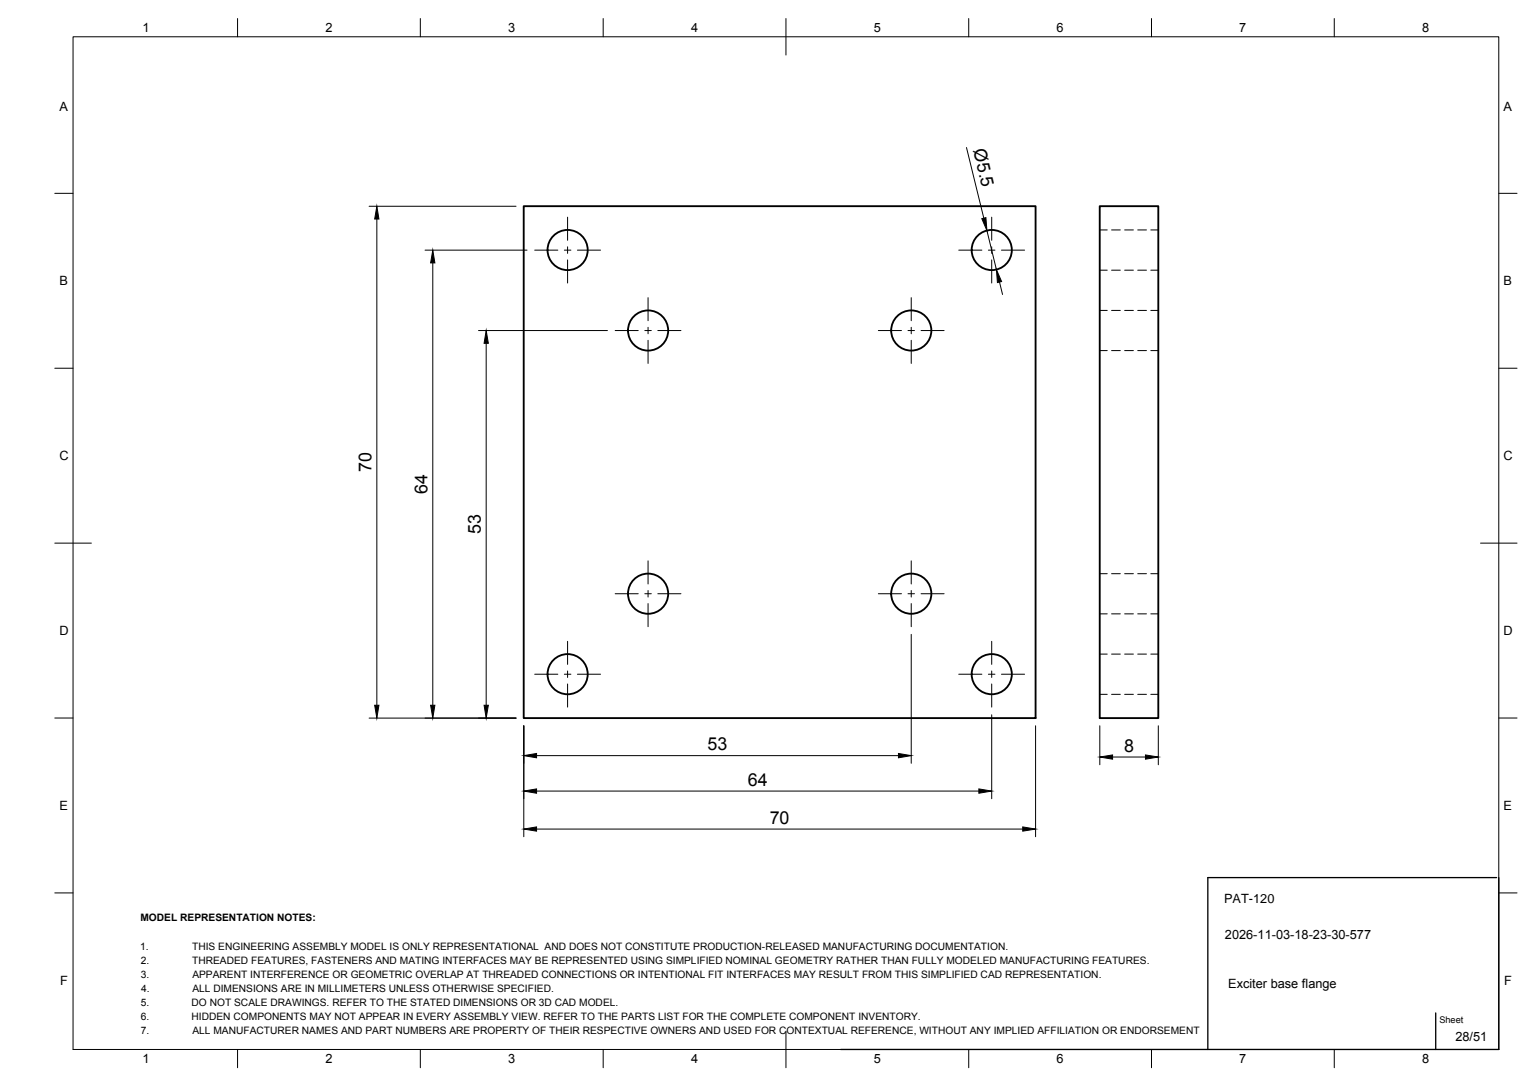
ISO-10303-21;
HEADER;
/* Generated by software containing ST-Developer
 * from STEP Tools, Inc. (www.steptools.com) 
 */

FILE_DESCRIPTION(
/* description */ ('Vibration shaker table dummy'),
/* implementation_level */ '2;1');

FILE_NAME(
/* name */ 'Exciter base flange.step',
/* time_stamp */ '2026-10-27T10:55:14-07:00',
/* author */ (''),
/* organization */ (''),
/* preprocessor_version */ 'ST-DEVELOPER v20.2',
/* originating_system */ 'Autodesk Translation Framework v15.17.0.0',
/* authorisation */ '');

FILE_SCHEMA (('AUTOMOTIVE_DESIGN { 1 0 10303 214 3 1 1 }'));
ENDSEC;

DATA;
#10=MECHANICAL_DESIGN_GEOMETRIC_PRESENTATION_REPRESENTATION('',(#709),#22394);
#617=SHAPE_REPRESENTATION_RELATIONSHIP('SRR','None',#22663,#663);
#663=ADVANCED_BREP_SHAPE_REPRESENTATION('',(#755),#22369);
#709=STYLED_ITEM('',(#22940),#755);
#755=MANIFOLD_SOLID_BREP('Body1',#9227);
#925=FACE_BOUND('',#2244,.T.);
#926=FACE_BOUND('',#2245,.T.);
#927=FACE_BOUND('',#2246,.T.);
#928=FACE_BOUND('',#2247,.T.);
#929=FACE_BOUND('',#2248,.T.);
#930=FACE_BOUND('',#2249,.T.);
#931=FACE_BOUND('',#2250,.T.);
#932=FACE_BOUND('',#2251,.T.);
#933=FACE_BOUND('',#2253,.T.);
#934=FACE_BOUND('',#2254,.T.);
#935=FACE_BOUND('',#2255,.T.);
#936=FACE_BOUND('',#2256,.T.);
#937=FACE_BOUND('',#2257,.T.);
#938=FACE_BOUND('',#2258,.T.);
#939=FACE_BOUND('',#2259,.T.);
#940=FACE_BOUND('',#2260,.T.);
#1204=PLANE('',#10260);
#1205=PLANE('',#10261);
#1206=PLANE('',#10262);
#1207=PLANE('',#10263);
#1208=PLANE('',#10264);
#1209=PLANE('',#10265);
#1583=FACE_OUTER_BOUND('',#2231,.T.);
#1584=FACE_OUTER_BOUND('',#2232,.T.);
#1585=FACE_OUTER_BOUND('',#2233,.T.);
#1586=FACE_OUTER_BOUND('',#2234,.T.);
#1587=FACE_OUTER_BOUND('',#2235,.T.);
#1588=FACE_OUTER_BOUND('',#2236,.T.);
#1589=FACE_OUTER_BOUND('',#2237,.T.);
#1590=FACE_OUTER_BOUND('',#2238,.T.);
#1591=FACE_OUTER_BOUND('',#2239,.T.);
#1592=FACE_OUTER_BOUND('',#2240,.T.);
#1593=FACE_OUTER_BOUND('',#2241,.T.);
#1594=FACE_OUTER_BOUND('',#2242,.T.);
#1595=FACE_OUTER_BOUND('',#2243,.T.);
#1596=FACE_OUTER_BOUND('',#2252,.T.);
#2231=EDGE_LOOP('',(#7338,#7339,#7340,#7341));
#2232=EDGE_LOOP('',(#7342,#7343,#7344,#7345));
#2233=EDGE_LOOP('',(#7346,#7347,#7348,#7349));
#2234=EDGE_LOOP('',(#7350,#7351,#7352,#7353));
#2235=EDGE_LOOP('',(#7354,#7355,#7356,#7357));
#2236=EDGE_LOOP('',(#7358,#7359,#7360,#7361));
#2237=EDGE_LOOP('',(#7362,#7363,#7364,#7365));
#2238=EDGE_LOOP('',(#7366,#7367,#7368,#7369));
#2239=EDGE_LOOP('',(#7370,#7371,#7372,#7373));
#2240=EDGE_LOOP('',(#7374,#7375,#7376,#7377));
#2241=EDGE_LOOP('',(#7378,#7379,#7380,#7381));
#2242=EDGE_LOOP('',(#7382,#7383,#7384,#7385));
#2243=EDGE_LOOP('',(#7386,#7387,#7388,#7389));
#2244=EDGE_LOOP('',(#7390));
#2245=EDGE_LOOP('',(#7391));
#2246=EDGE_LOOP('',(#7392));
#2247=EDGE_LOOP('',(#7393));
#2248=EDGE_LOOP('',(#7394));
#2249=EDGE_LOOP('',(#7395));
#2250=EDGE_LOOP('',(#7396));
#2251=EDGE_LOOP('',(#7397));
#2252=EDGE_LOOP('',(#7398,#7399,#7400,#7401));
#2253=EDGE_LOOP('',(#7402));
#2254=EDGE_LOOP('',(#7403));
#2255=EDGE_LOOP('',(#7404));
#2256=EDGE_LOOP('',(#7405));
#2257=EDGE_LOOP('',(#7406));
#2258=EDGE_LOOP('',(#7407));
#2259=EDGE_LOOP('',(#7408));
#2260=EDGE_LOOP('',(#7409));
#2952=LINE('',#20909,#3571);
#2953=LINE('',#20915,#3572);
#2954=LINE('',#20921,#3573);
#2955=LINE('',#20927,#3574);
#2956=LINE('',#20933,#3575);
#2957=LINE('',#20939,#3576);
#2958=LINE('',#20945,#3577);
#2959=LINE('',#20951,#3578);
#2960=LINE('',#20956,#3579);
#2961=LINE('',#20958,#3580);
#2962=LINE('',#20960,#3581);
#2963=LINE('',#20961,#3582);
#2964=LINE('',#20964,#3583);
#2965=LINE('',#20966,#3584);
#2966=LINE('',#20967,#3585);
#2967=LINE('',#20970,#3586);
#2968=LINE('',#20972,#3587);
#2969=LINE('',#20973,#3588);
#2970=LINE('',#20975,#3589);
#2971=LINE('',#20976,#3590);
#3571=VECTOR('',#12236,0.275);
#3572=VECTOR('',#12243,0.275);
#3573=VECTOR('',#12250,0.275);
#3574=VECTOR('',#12257,0.275);
#3575=VECTOR('',#12264,0.275);
#3576=VECTOR('',#12271,0.275);
#3577=VECTOR('',#12278,0.275);
#3578=VECTOR('',#12285,0.275);
#3579=VECTOR('',#12290,1.);
#3580=VECTOR('',#12291,1.);
#3581=VECTOR('',#12292,1.);
#3582=VECTOR('',#12293,1.);
#3583=VECTOR('',#12296,1.);
#3584=VECTOR('',#12297,1.);
#3585=VECTOR('',#12298,1.);
#3586=VECTOR('',#12301,1.);
#3587=VECTOR('',#12302,1.);
#3588=VECTOR('',#12303,1.);
#3589=VECTOR('',#12306,1.);
#3590=VECTOR('',#12307,1.);
#4072=CIRCLE('',#10237,0.275);
#4073=CIRCLE('',#10238,0.275);
#4074=CIRCLE('',#10240,0.275);
#4075=CIRCLE('',#10241,0.275);
#4076=CIRCLE('',#10243,0.275);
#4077=CIRCLE('',#10244,0.275);
#4078=CIRCLE('',#10246,0.275);
#4079=CIRCLE('',#10247,0.275);
#4080=CIRCLE('',#10249,0.275);
#4081=CIRCLE('',#10250,0.275);
#4082=CIRCLE('',#10252,0.275);
#4083=CIRCLE('',#10253,0.275);
#4084=CIRCLE('',#10255,0.275);
#4085=CIRCLE('',#10256,0.275);
#4086=CIRCLE('',#10258,0.275);
#4087=CIRCLE('',#10259,0.275);
#4731=VERTEX_POINT('',#20906);
#4732=VERTEX_POINT('',#20908);
#4733=VERTEX_POINT('',#20912);
#4734=VERTEX_POINT('',#20914);
#4735=VERTEX_POINT('',#20918);
#4736=VERTEX_POINT('',#20920);
#4737=VERTEX_POINT('',#20924);
#4738=VERTEX_POINT('',#20926);
#4739=VERTEX_POINT('',#20930);
#4740=VERTEX_POINT('',#20932);
#4741=VERTEX_POINT('',#20936);
#4742=VERTEX_POINT('',#20938);
#4743=VERTEX_POINT('',#20942);
#4744=VERTEX_POINT('',#20944);
#4745=VERTEX_POINT('',#20948);
#4746=VERTEX_POINT('',#20950);
#4747=VERTEX_POINT('',#20954);
#4748=VERTEX_POINT('',#20955);
#4749=VERTEX_POINT('',#20957);
#4750=VERTEX_POINT('',#20959);
#4751=VERTEX_POINT('',#20963);
#4752=VERTEX_POINT('',#20965);
#4753=VERTEX_POINT('',#20969);
#4754=VERTEX_POINT('',#20971);
#5662=EDGE_CURVE('',#4731,#4731,#4072,.T.);
#5663=EDGE_CURVE('',#4731,#4732,#2952,.T.);
#5664=EDGE_CURVE('',#4732,#4732,#4073,.T.);
#5665=EDGE_CURVE('',#4733,#4733,#4074,.T.);
#5666=EDGE_CURVE('',#4733,#4734,#2953,.T.);
#5667=EDGE_CURVE('',#4734,#4734,#4075,.T.);
#5668=EDGE_CURVE('',#4735,#4735,#4076,.T.);
#5669=EDGE_CURVE('',#4735,#4736,#2954,.T.);
#5670=EDGE_CURVE('',#4736,#4736,#4077,.T.);
#5671=EDGE_CURVE('',#4737,#4737,#4078,.T.);
#5672=EDGE_CURVE('',#4737,#4738,#2955,.T.);
#5673=EDGE_CURVE('',#4738,#4738,#4079,.T.);
#5674=EDGE_CURVE('',#4739,#4739,#4080,.T.);
#5675=EDGE_CURVE('',#4739,#4740,#2956,.T.);
#5676=EDGE_CURVE('',#4740,#4740,#4081,.T.);
#5677=EDGE_CURVE('',#4741,#4741,#4082,.T.);
#5678=EDGE_CURVE('',#4741,#4742,#2957,.T.);
#5679=EDGE_CURVE('',#4742,#4742,#4083,.T.);
#5680=EDGE_CURVE('',#4743,#4743,#4084,.T.);
#5681=EDGE_CURVE('',#4743,#4744,#2958,.T.);
#5682=EDGE_CURVE('',#4744,#4744,#4085,.T.);
#5683=EDGE_CURVE('',#4745,#4745,#4086,.T.);
#5684=EDGE_CURVE('',#4745,#4746,#2959,.T.);
#5685=EDGE_CURVE('',#4746,#4746,#4087,.T.);
#5686=EDGE_CURVE('',#4747,#4748,#2960,.T.);
#5687=EDGE_CURVE('',#4748,#4749,#2961,.T.);
#5688=EDGE_CURVE('',#4750,#4749,#2962,.T.);
#5689=EDGE_CURVE('',#4747,#4750,#2963,.T.);
#5690=EDGE_CURVE('',#4751,#4747,#2964,.T.);
#5691=EDGE_CURVE('',#4752,#4750,#2965,.T.);
#5692=EDGE_CURVE('',#4751,#4752,#2966,.T.);
#5693=EDGE_CURVE('',#4753,#4751,#2967,.T.);
#5694=EDGE_CURVE('',#4754,#4752,#2968,.T.);
#5695=EDGE_CURVE('',#4753,#4754,#2969,.T.);
#5696=EDGE_CURVE('',#4748,#4753,#2970,.T.);
#5697=EDGE_CURVE('',#4749,#4754,#2971,.T.);
#7338=ORIENTED_EDGE('',*,*,#5662,.F.);
#7339=ORIENTED_EDGE('',*,*,#5663,.T.);
#7340=ORIENTED_EDGE('',*,*,#5664,.F.);
#7341=ORIENTED_EDGE('',*,*,#5663,.F.);
#7342=ORIENTED_EDGE('',*,*,#5665,.F.);
#7343=ORIENTED_EDGE('',*,*,#5666,.T.);
#7344=ORIENTED_EDGE('',*,*,#5667,.F.);
#7345=ORIENTED_EDGE('',*,*,#5666,.F.);
#7346=ORIENTED_EDGE('',*,*,#5668,.F.);
#7347=ORIENTED_EDGE('',*,*,#5669,.T.);
#7348=ORIENTED_EDGE('',*,*,#5670,.F.);
#7349=ORIENTED_EDGE('',*,*,#5669,.F.);
#7350=ORIENTED_EDGE('',*,*,#5671,.F.);
#7351=ORIENTED_EDGE('',*,*,#5672,.T.);
#7352=ORIENTED_EDGE('',*,*,#5673,.F.);
#7353=ORIENTED_EDGE('',*,*,#5672,.F.);
#7354=ORIENTED_EDGE('',*,*,#5674,.F.);
#7355=ORIENTED_EDGE('',*,*,#5675,.T.);
#7356=ORIENTED_EDGE('',*,*,#5676,.F.);
#7357=ORIENTED_EDGE('',*,*,#5675,.F.);
#7358=ORIENTED_EDGE('',*,*,#5677,.F.);
#7359=ORIENTED_EDGE('',*,*,#5678,.T.);
#7360=ORIENTED_EDGE('',*,*,#5679,.F.);
#7361=ORIENTED_EDGE('',*,*,#5678,.F.);
#7362=ORIENTED_EDGE('',*,*,#5680,.F.);
#7363=ORIENTED_EDGE('',*,*,#5681,.T.);
#7364=ORIENTED_EDGE('',*,*,#5682,.F.);
#7365=ORIENTED_EDGE('',*,*,#5681,.F.);
#7366=ORIENTED_EDGE('',*,*,#5683,.F.);
#7367=ORIENTED_EDGE('',*,*,#5684,.T.);
#7368=ORIENTED_EDGE('',*,*,#5685,.F.);
#7369=ORIENTED_EDGE('',*,*,#5684,.F.);
#7370=ORIENTED_EDGE('',*,*,#5686,.T.);
#7371=ORIENTED_EDGE('',*,*,#5687,.T.);
#7372=ORIENTED_EDGE('',*,*,#5688,.F.);
#7373=ORIENTED_EDGE('',*,*,#5689,.F.);
#7374=ORIENTED_EDGE('',*,*,#5690,.T.);
#7375=ORIENTED_EDGE('',*,*,#5689,.T.);
#7376=ORIENTED_EDGE('',*,*,#5691,.F.);
#7377=ORIENTED_EDGE('',*,*,#5692,.F.);
#7378=ORIENTED_EDGE('',*,*,#5693,.T.);
#7379=ORIENTED_EDGE('',*,*,#5692,.T.);
#7380=ORIENTED_EDGE('',*,*,#5694,.F.);
#7381=ORIENTED_EDGE('',*,*,#5695,.F.);
#7382=ORIENTED_EDGE('',*,*,#5696,.T.);
#7383=ORIENTED_EDGE('',*,*,#5695,.T.);
#7384=ORIENTED_EDGE('',*,*,#5697,.F.);
#7385=ORIENTED_EDGE('',*,*,#5687,.F.);
#7386=ORIENTED_EDGE('',*,*,#5697,.T.);
#7387=ORIENTED_EDGE('',*,*,#5694,.T.);
#7388=ORIENTED_EDGE('',*,*,#5691,.T.);
#7389=ORIENTED_EDGE('',*,*,#5688,.T.);
#7390=ORIENTED_EDGE('',*,*,#5685,.T.);
#7391=ORIENTED_EDGE('',*,*,#5682,.T.);
#7392=ORIENTED_EDGE('',*,*,#5679,.T.);
#7393=ORIENTED_EDGE('',*,*,#5676,.T.);
#7394=ORIENTED_EDGE('',*,*,#5673,.T.);
#7395=ORIENTED_EDGE('',*,*,#5670,.T.);
#7396=ORIENTED_EDGE('',*,*,#5667,.T.);
#7397=ORIENTED_EDGE('',*,*,#5664,.T.);
#7398=ORIENTED_EDGE('',*,*,#5696,.F.);
#7399=ORIENTED_EDGE('',*,*,#5686,.F.);
#7400=ORIENTED_EDGE('',*,*,#5690,.F.);
#7401=ORIENTED_EDGE('',*,*,#5693,.F.);
#7402=ORIENTED_EDGE('',*,*,#5683,.T.);
#7403=ORIENTED_EDGE('',*,*,#5680,.T.);
#7404=ORIENTED_EDGE('',*,*,#5677,.T.);
#7405=ORIENTED_EDGE('',*,*,#5674,.T.);
#7406=ORIENTED_EDGE('',*,*,#5671,.T.);
#7407=ORIENTED_EDGE('',*,*,#5668,.T.);
#7408=ORIENTED_EDGE('',*,*,#5665,.T.);
#7409=ORIENTED_EDGE('',*,*,#5662,.T.);
#8600=CYLINDRICAL_SURFACE('',#10236,0.275);
#8601=CYLINDRICAL_SURFACE('',#10239,0.275);
#8602=CYLINDRICAL_SURFACE('',#10242,0.275);
#8603=CYLINDRICAL_SURFACE('',#10245,0.275);
#8604=CYLINDRICAL_SURFACE('',#10248,0.275);
#8605=CYLINDRICAL_SURFACE('',#10251,0.275);
#8606=CYLINDRICAL_SURFACE('',#10254,0.275);
#8607=CYLINDRICAL_SURFACE('',#10257,0.275);
#8948=ADVANCED_FACE('',(#1583),#8600,.F.);
#8949=ADVANCED_FACE('',(#1584),#8601,.F.);
#8950=ADVANCED_FACE('',(#1585),#8602,.F.);
#8951=ADVANCED_FACE('',(#1586),#8603,.F.);
#8952=ADVANCED_FACE('',(#1587),#8604,.F.);
#8953=ADVANCED_FACE('',(#1588),#8605,.F.);
#8954=ADVANCED_FACE('',(#1589),#8606,.F.);
#8955=ADVANCED_FACE('',(#1590),#8607,.F.);
#8956=ADVANCED_FACE('',(#1591),#1204,.T.);
#8957=ADVANCED_FACE('',(#1592),#1205,.T.);
#8958=ADVANCED_FACE('',(#1593),#1206,.T.);
#8959=ADVANCED_FACE('',(#1594),#1207,.T.);
#8960=ADVANCED_FACE('',(#1595,#925,#926,#927,#928,#929,#930,#931,#932),
#1208,.T.);
#8961=ADVANCED_FACE('',(#1596,#933,#934,#935,#936,#937,#938,#939,#940),
#1209,.F.);
#9227=CLOSED_SHELL('',(#8948,#8949,#8950,#8951,#8952,#8953,#8954,#8955,
#8956,#8957,#8958,#8959,#8960,#8961));
#10235=AXIS2_PLACEMENT_3D('',#20904,#12230,#12231);
#10236=AXIS2_PLACEMENT_3D('',#20905,#12232,#12233);
#10237=AXIS2_PLACEMENT_3D('',#20907,#12234,#12235);
#10238=AXIS2_PLACEMENT_3D('',#20910,#12237,#12238);
#10239=AXIS2_PLACEMENT_3D('',#20911,#12239,#12240);
#10240=AXIS2_PLACEMENT_3D('',#20913,#12241,#12242);
#10241=AXIS2_PLACEMENT_3D('',#20916,#12244,#12245);
#10242=AXIS2_PLACEMENT_3D('',#20917,#12246,#12247);
#10243=AXIS2_PLACEMENT_3D('',#20919,#12248,#12249);
#10244=AXIS2_PLACEMENT_3D('',#20922,#12251,#12252);
#10245=AXIS2_PLACEMENT_3D('',#20923,#12253,#12254);
#10246=AXIS2_PLACEMENT_3D('',#20925,#12255,#12256);
#10247=AXIS2_PLACEMENT_3D('',#20928,#12258,#12259);
#10248=AXIS2_PLACEMENT_3D('',#20929,#12260,#12261);
#10249=AXIS2_PLACEMENT_3D('',#20931,#12262,#12263);
#10250=AXIS2_PLACEMENT_3D('',#20934,#12265,#12266);
#10251=AXIS2_PLACEMENT_3D('',#20935,#12267,#12268);
#10252=AXIS2_PLACEMENT_3D('',#20937,#12269,#12270);
#10253=AXIS2_PLACEMENT_3D('',#20940,#12272,#12273);
#10254=AXIS2_PLACEMENT_3D('',#20941,#12274,#12275);
#10255=AXIS2_PLACEMENT_3D('',#20943,#12276,#12277);
#10256=AXIS2_PLACEMENT_3D('',#20946,#12279,#12280);
#10257=AXIS2_PLACEMENT_3D('',#20947,#12281,#12282);
#10258=AXIS2_PLACEMENT_3D('',#20949,#12283,#12284);
#10259=AXIS2_PLACEMENT_3D('',#20952,#12286,#12287);
#10260=AXIS2_PLACEMENT_3D('',#20953,#12288,#12289);
#10261=AXIS2_PLACEMENT_3D('',#20962,#12294,#12295);
#10262=AXIS2_PLACEMENT_3D('',#20968,#12299,#12300);
#10263=AXIS2_PLACEMENT_3D('',#20974,#12304,#12305);
#10264=AXIS2_PLACEMENT_3D('',#20977,#12308,#12309);
#10265=AXIS2_PLACEMENT_3D('',#20978,#12310,#12311);
#12230=DIRECTION('axis',(0.,0.,1.));
#12231=DIRECTION('refdir',(1.,0.,0.));
#12232=DIRECTION('center_axis',(0.,0.,1.));
#12233=DIRECTION('ref_axis',(1.,0.,0.));
#12234=DIRECTION('center_axis',(0.,0.,1.));
#12235=DIRECTION('ref_axis',(1.,0.,0.));
#12236=DIRECTION('',(0.,0.,1.));
#12237=DIRECTION('center_axis',(0.,0.,-1.));
#12238=DIRECTION('ref_axis',(1.,0.,0.));
#12239=DIRECTION('center_axis',(0.,0.,1.));
#12240=DIRECTION('ref_axis',(1.,0.,0.));
#12241=DIRECTION('center_axis',(0.,0.,1.));
#12242=DIRECTION('ref_axis',(1.,0.,0.));
#12243=DIRECTION('',(0.,0.,1.));
#12244=DIRECTION('center_axis',(0.,0.,-1.));
#12245=DIRECTION('ref_axis',(1.,0.,0.));
#12246=DIRECTION('center_axis',(0.,0.,1.));
#12247=DIRECTION('ref_axis',(1.,0.,0.));
#12248=DIRECTION('center_axis',(0.,0.,1.));
#12249=DIRECTION('ref_axis',(1.,0.,0.));
#12250=DIRECTION('',(0.,0.,1.));
#12251=DIRECTION('center_axis',(0.,0.,-1.));
#12252=DIRECTION('ref_axis',(1.,0.,0.));
#12253=DIRECTION('center_axis',(0.,0.,1.));
#12254=DIRECTION('ref_axis',(1.,0.,0.));
#12255=DIRECTION('center_axis',(0.,0.,1.));
#12256=DIRECTION('ref_axis',(1.,0.,0.));
#12257=DIRECTION('',(0.,0.,1.));
#12258=DIRECTION('center_axis',(0.,0.,-1.));
#12259=DIRECTION('ref_axis',(1.,0.,0.));
#12260=DIRECTION('center_axis',(0.,0.,1.));
#12261=DIRECTION('ref_axis',(1.,0.,0.));
#12262=DIRECTION('center_axis',(0.,0.,1.));
#12263=DIRECTION('ref_axis',(1.,0.,0.));
#12264=DIRECTION('',(0.,0.,1.));
#12265=DIRECTION('center_axis',(0.,0.,-1.));
#12266=DIRECTION('ref_axis',(1.,0.,0.));
#12267=DIRECTION('center_axis',(0.,0.,1.));
#12268=DIRECTION('ref_axis',(1.,0.,0.));
#12269=DIRECTION('center_axis',(0.,0.,1.));
#12270=DIRECTION('ref_axis',(1.,0.,0.));
#12271=DIRECTION('',(0.,0.,1.));
#12272=DIRECTION('center_axis',(0.,0.,-1.));
#12273=DIRECTION('ref_axis',(1.,0.,0.));
#12274=DIRECTION('center_axis',(0.,0.,1.));
#12275=DIRECTION('ref_axis',(1.,0.,0.));
#12276=DIRECTION('center_axis',(0.,0.,1.));
#12277=DIRECTION('ref_axis',(1.,0.,0.));
#12278=DIRECTION('',(0.,0.,1.));
#12279=DIRECTION('center_axis',(0.,0.,-1.));
#12280=DIRECTION('ref_axis',(1.,0.,0.));
#12281=DIRECTION('center_axis',(0.,0.,1.));
#12282=DIRECTION('ref_axis',(1.,0.,0.));
#12283=DIRECTION('center_axis',(0.,0.,1.));
#12284=DIRECTION('ref_axis',(1.,0.,0.));
#12285=DIRECTION('',(0.,0.,1.));
#12286=DIRECTION('center_axis',(0.,0.,-1.));
#12287=DIRECTION('ref_axis',(1.,0.,0.));
#12288=DIRECTION('center_axis',(0.,1.,0.));
#12289=DIRECTION('ref_axis',(-1.,0.,0.));
#12290=DIRECTION('',(-1.,0.,0.));
#12291=DIRECTION('',(0.,0.,1.));
#12292=DIRECTION('',(-1.,0.,0.));
#12293=DIRECTION('',(0.,0.,1.));
#12294=DIRECTION('center_axis',(1.,0.,0.));
#12295=DIRECTION('ref_axis',(0.,1.,0.));
#12296=DIRECTION('',(0.,1.,0.));
#12297=DIRECTION('',(0.,1.,0.));
#12298=DIRECTION('',(0.,0.,1.));
#12299=DIRECTION('center_axis',(0.,-1.,0.));
#12300=DIRECTION('ref_axis',(1.,0.,0.));
#12301=DIRECTION('',(1.,0.,0.));
#12302=DIRECTION('',(1.,0.,0.));
#12303=DIRECTION('',(0.,0.,1.));
#12304=DIRECTION('center_axis',(-1.,0.,0.));
#12305=DIRECTION('ref_axis',(0.,-1.,0.));
#12306=DIRECTION('',(0.,-1.,0.));
#12307=DIRECTION('',(0.,-1.,0.));
#12308=DIRECTION('center_axis',(0.,0.,1.));
#12309=DIRECTION('ref_axis',(1.,0.,0.));
#12310=DIRECTION('center_axis',(0.,0.,1.));
#12311=DIRECTION('ref_axis',(1.,0.,0.));
#20904=CARTESIAN_POINT('',(0.,0.,0.));
#20905=CARTESIAN_POINT('Origin',(1.8,-1.8,-0.1));
#20906=CARTESIAN_POINT('',(1.525,-1.8,0.));
#20907=CARTESIAN_POINT('Origin',(1.8,-1.8,0.));
#20908=CARTESIAN_POINT('',(1.525,-1.8,0.8));
#20909=CARTESIAN_POINT('',(1.525,-1.8,-0.1));
#20910=CARTESIAN_POINT('Origin',(1.8,-1.8,0.8));
#20911=CARTESIAN_POINT('Origin',(-1.8,1.8,-0.1));
#20912=CARTESIAN_POINT('',(-2.075,1.8,0.));
#20913=CARTESIAN_POINT('Origin',(-1.8,1.8,0.));
#20914=CARTESIAN_POINT('',(-2.075,1.8,0.8));
#20915=CARTESIAN_POINT('',(-2.075,1.8,-0.1));
#20916=CARTESIAN_POINT('Origin',(-1.8,1.8,0.8));
#20917=CARTESIAN_POINT('Origin',(-1.8,-1.8,-0.1));
#20918=CARTESIAN_POINT('',(-2.075,-1.8,0.));
#20919=CARTESIAN_POINT('Origin',(-1.8,-1.8,0.));
#20920=CARTESIAN_POINT('',(-2.075,-1.8,0.8));
#20921=CARTESIAN_POINT('',(-2.075,-1.8,-0.1));
#20922=CARTESIAN_POINT('Origin',(-1.8,-1.8,0.8));
#20923=CARTESIAN_POINT('Origin',(1.8,1.8,-0.1));
#20924=CARTESIAN_POINT('',(1.525,1.8,0.));
#20925=CARTESIAN_POINT('Origin',(1.8,1.8,0.));
#20926=CARTESIAN_POINT('',(1.525,1.8,0.8));
#20927=CARTESIAN_POINT('',(1.525,1.8,-0.1));
#20928=CARTESIAN_POINT('Origin',(1.8,1.8,0.8));
#20929=CARTESIAN_POINT('Origin',(2.9,-2.9,-0.1));
#20930=CARTESIAN_POINT('',(2.625,-2.9,0.));
#20931=CARTESIAN_POINT('Origin',(2.9,-2.9,0.));
#20932=CARTESIAN_POINT('',(2.625,-2.9,0.8));
#20933=CARTESIAN_POINT('',(2.625,-2.9,-0.1));
#20934=CARTESIAN_POINT('Origin',(2.9,-2.9,0.8));
#20935=CARTESIAN_POINT('Origin',(-2.9,2.9,-0.1));
#20936=CARTESIAN_POINT('',(-3.175,2.9,0.));
#20937=CARTESIAN_POINT('Origin',(-2.9,2.9,0.));
#20938=CARTESIAN_POINT('',(-3.175,2.9,0.8));
#20939=CARTESIAN_POINT('',(-3.175,2.9,-0.1));
#20940=CARTESIAN_POINT('Origin',(-2.9,2.9,0.8));
#20941=CARTESIAN_POINT('Origin',(-2.9,-2.9,-0.1));
#20942=CARTESIAN_POINT('',(-3.175,-2.9,0.));
#20943=CARTESIAN_POINT('Origin',(-2.9,-2.9,0.));
#20944=CARTESIAN_POINT('',(-3.175,-2.9,0.8));
#20945=CARTESIAN_POINT('',(-3.175,-2.9,-0.1));
#20946=CARTESIAN_POINT('Origin',(-2.9,-2.9,0.8));
#20947=CARTESIAN_POINT('Origin',(2.9,2.9,-0.1));
#20948=CARTESIAN_POINT('',(2.625,2.9,0.));
#20949=CARTESIAN_POINT('Origin',(2.9,2.9,0.));
#20950=CARTESIAN_POINT('',(2.625,2.9,0.8));
#20951=CARTESIAN_POINT('',(2.625,2.9,-0.1));
#20952=CARTESIAN_POINT('Origin',(2.9,2.9,0.8));
#20953=CARTESIAN_POINT('Origin',(3.5,3.5,0.));
#20954=CARTESIAN_POINT('',(3.5,3.5,0.));
#20955=CARTESIAN_POINT('',(-3.5,3.5,0.));
#20956=CARTESIAN_POINT('',(3.5,3.5,0.));
#20957=CARTESIAN_POINT('',(-3.5,3.5,0.8));
#20958=CARTESIAN_POINT('',(-3.5,3.5,0.));
#20959=CARTESIAN_POINT('',(3.5,3.5,0.8));
#20960=CARTESIAN_POINT('',(3.5,3.5,0.8));
#20961=CARTESIAN_POINT('',(3.5,3.5,0.));
#20962=CARTESIAN_POINT('Origin',(3.5,-3.5,0.));
#20963=CARTESIAN_POINT('',(3.5,-3.5,0.));
#20964=CARTESIAN_POINT('',(3.5,-3.5,0.));
#20965=CARTESIAN_POINT('',(3.5,-3.5,0.8));
#20966=CARTESIAN_POINT('',(3.5,-3.5,0.8));
#20967=CARTESIAN_POINT('',(3.5,-3.5,0.));
#20968=CARTESIAN_POINT('Origin',(-3.5,-3.5,0.));
#20969=CARTESIAN_POINT('',(-3.5,-3.5,0.));
#20970=CARTESIAN_POINT('',(-3.5,-3.5,0.));
#20971=CARTESIAN_POINT('',(-3.5,-3.5,0.8));
#20972=CARTESIAN_POINT('',(-3.5,-3.5,0.8));
#20973=CARTESIAN_POINT('',(-3.5,-3.5,0.));
#20974=CARTESIAN_POINT('Origin',(-3.5,3.5,0.));
#20975=CARTESIAN_POINT('',(-3.5,3.5,0.));
#20976=CARTESIAN_POINT('',(-3.5,3.5,0.8));
#20977=CARTESIAN_POINT('Origin',(0.,0.,0.8));
#20978=CARTESIAN_POINT('Origin',(0.,0.,0.));
#22318=UNCERTAINTY_MEASURE_WITH_UNIT(LENGTH_MEASURE(0.001),#22395,
'DISTANCE_ACCURACY_VALUE',
'Maximum model space distance between geometric entities at asserted c
onnectivities');
#22343=UNCERTAINTY_MEASURE_WITH_UNIT(LENGTH_MEASURE(0.001),#22395,
'DISTANCE_ACCURACY_VALUE',
'Maximum model space distance between geometric entities at asserted c
onnectivities');
#22369=(
GEOMETRIC_REPRESENTATION_CONTEXT(3)
GLOBAL_UNCERTAINTY_ASSIGNED_CONTEXT((#22318))
GLOBAL_UNIT_ASSIGNED_CONTEXT((#22395,#22397,#22398))
REPRESENTATION_CONTEXT('','3D')
);
#22394=(
GEOMETRIC_REPRESENTATION_CONTEXT(3)
GLOBAL_UNCERTAINTY_ASSIGNED_CONTEXT((#22343))
GLOBAL_UNIT_ASSIGNED_CONTEXT((#22395,#22397,#22398))
REPRESENTATION_CONTEXT('','3D')
);
#22395=(
LENGTH_UNIT()
NAMED_UNIT(*)
SI_UNIT(.CENTI.,.METRE.)
);
#22397=(
NAMED_UNIT(*)
PLANE_ANGLE_UNIT()
SI_UNIT($,.RADIAN.)
);
#22398=(
NAMED_UNIT(*)
SI_UNIT($,.STERADIAN.)
SOLID_ANGLE_UNIT()
);
#22424=SHAPE_DEFINITION_REPRESENTATION(#22474,#22663);
#22474=PRODUCT_DEFINITION_SHAPE('',$,#22714);
#22663=SHAPE_REPRESENTATION('',(#10235),#22369);
#22688=PRODUCT_DEFINITION_CONTEXT('part definition',#22840,'design');
#22714=PRODUCT_DEFINITION('Exciter base flange','Exciter base flange',#22764,
#22688);
#22764=PRODUCT_DEFINITION_FORMATION('',$,#22867);
#22840=APPLICATION_CONTEXT(
'Core Data for Automotive Mechanical Design Process');
#22841=PRODUCT_CONTEXT('part definition',#22840,'mechanical');
#22867=PRODUCT('Exciter base flange','Exciter base flange',
'Exciter base flange',(#22841));
#22934=COLOUR_RGB('Dark Blue',0.08,0.2,0.34);
#22935=FILL_AREA_STYLE_COLOUR('',#22934);
#22936=FILL_AREA_STYLE('',(#22935));
#22937=SURFACE_STYLE_FILL_AREA(#22936);
#22938=SURFACE_SIDE_STYLE('',(#22937));
#22939=SURFACE_STYLE_USAGE(.BOTH.,#22938);
#22940=PRESENTATION_STYLE_ASSIGNMENT((#22939));
ENDSEC;
END-ISO-10303-21;
